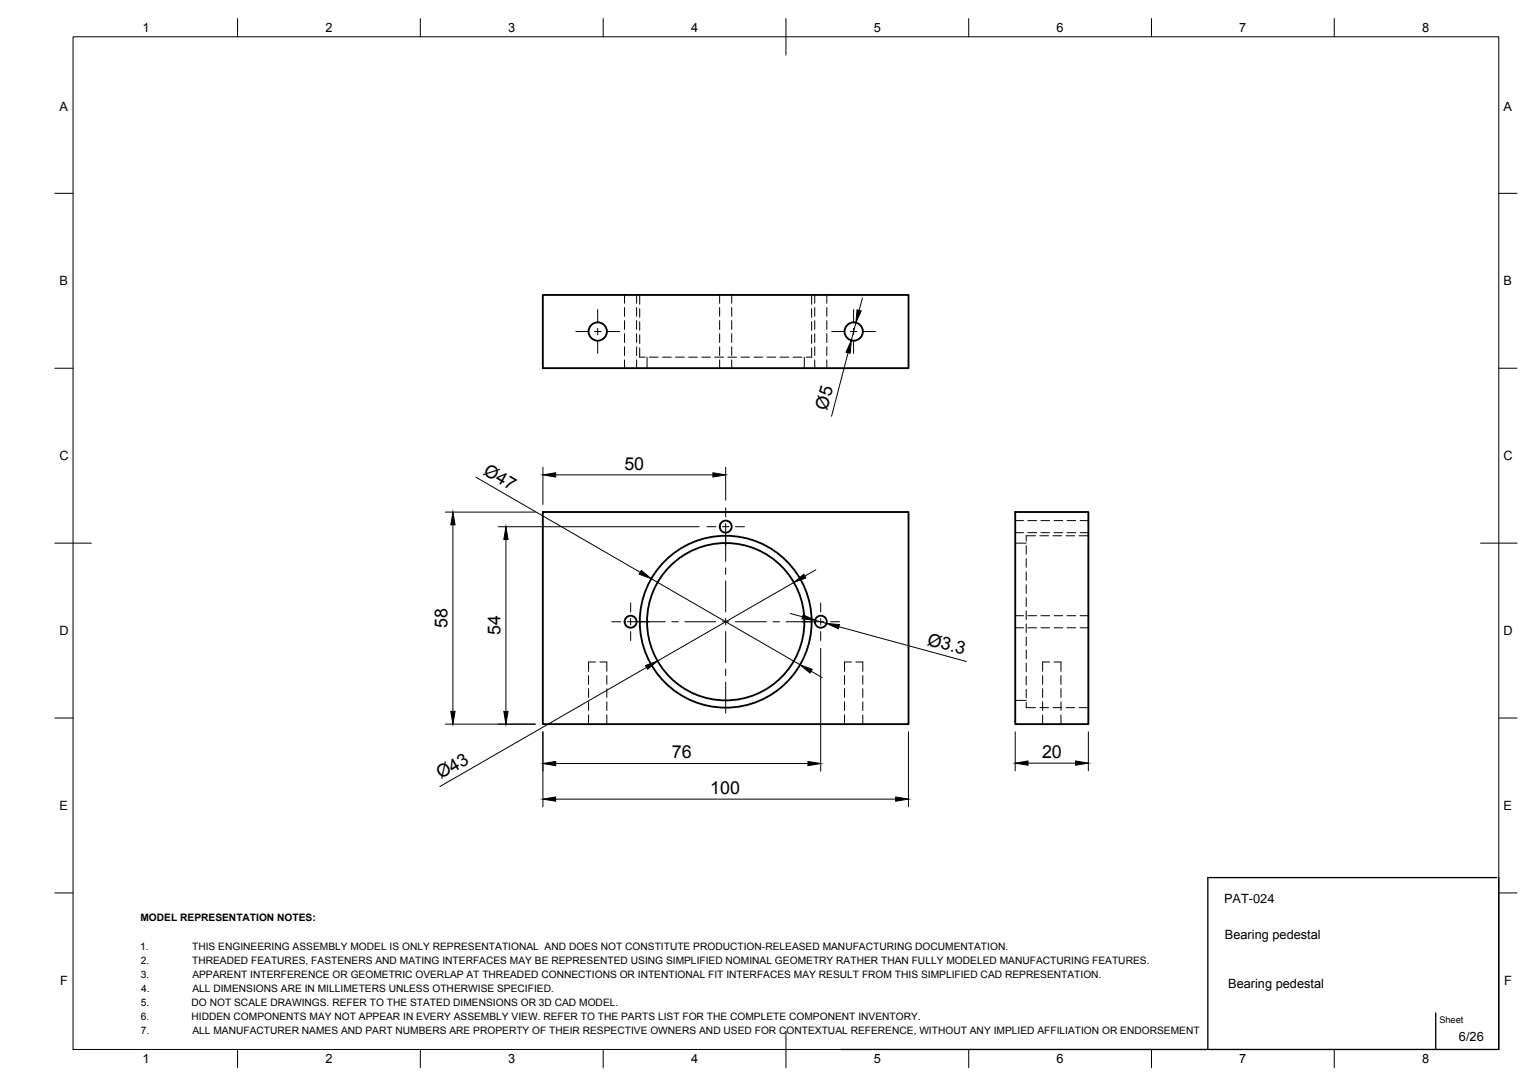
ISO-10303-21;
HEADER;
/* Generated by software containing ST-Developer
 * from STEP Tools, Inc. (www.steptools.com) 
 */

FILE_DESCRIPTION(
/* description */ ('Compact handwheel screw vise'),
/* implementation_level */ '2;1');

FILE_NAME(
/* name */ 'Bearing pedestal.step',
/* time_stamp */ '2026-10-29T16:08:22-07:00',
/* author */ (''),
/* organization */ (''),
/* preprocessor_version */ 'ST-DEVELOPER v20.2',
/* originating_system */ 'Autodesk Translation Framework v15.17.0.0',
/* authorisation */ '');

FILE_SCHEMA (('AUTOMOTIVE_DESIGN { 1 0 10303 214 3 1 1 }'));
ENDSEC;

DATA;
#10=MECHANICAL_DESIGN_GEOMETRIC_PRESENTATION_REPRESENTATION('',(#647),#25074);
#591=SHAPE_REPRESENTATION_RELATIONSHIP('SRR','None',#25199,#619);
#619=ADVANCED_BREP_SHAPE_REPRESENTATION('',(#683),#25046);
#647=STYLED_ITEM('',(#25439),#683);
#683=MANIFOLD_SOLID_BREP('Body1',#8055);
#733=FACE_BOUND('',#1547,.T.);
#734=FACE_BOUND('',#1555,.T.);
#735=FACE_BOUND('',#1556,.T.);
#736=FACE_BOUND('',#1557,.T.);
#737=FACE_BOUND('',#1558,.T.);
#738=FACE_BOUND('',#1561,.T.);
#739=FACE_BOUND('',#1562,.T.);
#740=FACE_BOUND('',#1563,.T.);
#741=FACE_BOUND('',#1564,.T.);
#742=FACE_BOUND('',#1567,.T.);
#743=FACE_BOUND('',#1568,.T.);
#847=PLANE('',#8486);
#848=PLANE('',#8493);
#849=PLANE('',#8497);
#850=PLANE('',#8498);
#851=PLANE('',#8499);
#852=PLANE('',#8500);
#853=PLANE('',#8501);
#854=PLANE('',#8502);
#855=PLANE('',#8503);
#1051=FACE_OUTER_BOUND('',#1542,.T.);
#1052=FACE_OUTER_BOUND('',#1543,.T.);
#1053=FACE_OUTER_BOUND('',#1544,.T.);
#1054=FACE_OUTER_BOUND('',#1545,.T.);
#1055=FACE_OUTER_BOUND('',#1546,.T.);
#1056=FACE_OUTER_BOUND('',#1548,.T.);
#1057=FACE_OUTER_BOUND('',#1549,.T.);
#1058=FACE_OUTER_BOUND('',#1550,.T.);
#1059=FACE_OUTER_BOUND('',#1551,.T.);
#1060=FACE_OUTER_BOUND('',#1552,.T.);
#1061=FACE_OUTER_BOUND('',#1553,.T.);
#1062=FACE_OUTER_BOUND('',#1554,.T.);
#1063=FACE_OUTER_BOUND('',#1559,.T.);
#1064=FACE_OUTER_BOUND('',#1560,.T.);
#1065=FACE_OUTER_BOUND('',#1565,.T.);
#1066=FACE_OUTER_BOUND('',#1566,.T.);
#1542=EDGE_LOOP('',(#5315,#5316,#5317,#5318));
#1543=EDGE_LOOP('',(#5319,#5320,#5321,#5322));
#1544=EDGE_LOOP('',(#5323,#5324,#5325,#5326));
#1545=EDGE_LOOP('',(#5327,#5328,#5329,#5330));
#1546=EDGE_LOOP('',(#5331));
#1547=EDGE_LOOP('',(#5332));
#1548=EDGE_LOOP('',(#5333,#5334,#5335,#5336));
#1549=EDGE_LOOP('',(#5337,#5338,#5339,#5340));
#1550=EDGE_LOOP('',(#5341));
#1551=EDGE_LOOP('',(#5342,#5343,#5344,#5345));
#1552=EDGE_LOOP('',(#5346));
#1553=EDGE_LOOP('',(#5347,#5348,#5349,#5350));
#1554=EDGE_LOOP('',(#5351,#5352,#5353,#5354));
#1555=EDGE_LOOP('',(#5355));
#1556=EDGE_LOOP('',(#5356));
#1557=EDGE_LOOP('',(#5357));
#1558=EDGE_LOOP('',(#5358));
#1559=EDGE_LOOP('',(#5359,#5360,#5361,#5362));
#1560=EDGE_LOOP('',(#5363,#5364,#5365,#5366));
#1561=EDGE_LOOP('',(#5367));
#1562=EDGE_LOOP('',(#5368));
#1563=EDGE_LOOP('',(#5369));
#1564=EDGE_LOOP('',(#5370));
#1565=EDGE_LOOP('',(#5371,#5372,#5373,#5374));
#1566=EDGE_LOOP('',(#5375,#5376,#5377,#5378));
#1567=EDGE_LOOP('',(#5379));
#1568=EDGE_LOOP('',(#5380));
#2112=LINE('',#11497,#2620);
#2113=LINE('',#11503,#2621);
#2114=LINE('',#11509,#2622);
#2115=LINE('',#11515,#2623);
#2116=LINE('',#11523,#2624);
#2117=LINE('',#11528,#2625);
#2118=LINE('',#11535,#2626);
#2119=LINE('',#11541,#2627);
#2120=LINE('',#11543,#2628);
#2121=LINE('',#11545,#2629);
#2122=LINE('',#11546,#2630);
#2123=LINE('',#11549,#2631);
#2124=LINE('',#11551,#2632);
#2125=LINE('',#11552,#2633);
#2126=LINE('',#11555,#2634);
#2127=LINE('',#11557,#2635);
#2128=LINE('',#11558,#2636);
#2129=LINE('',#11560,#2637);
#2130=LINE('',#11561,#2638);
#2620=VECTOR('',#9404,0.165);
#2621=VECTOR('',#9411,0.165);
#2622=VECTOR('',#9418,0.165);
#2623=VECTOR('',#9425,2.35);
#2624=VECTOR('',#9436,2.15);
#2625=VECTOR('',#9441,0.25);
#2626=VECTOR('',#9450,0.25);
#2627=VECTOR('',#9457,1.);
#2628=VECTOR('',#9458,1.);
#2629=VECTOR('',#9459,1.);
#2630=VECTOR('',#9460,1.);
#2631=VECTOR('',#9463,1.);
#2632=VECTOR('',#9464,1.);
#2633=VECTOR('',#9465,1.);
#2634=VECTOR('',#9468,1.);
#2635=VECTOR('',#9469,1.);
#2636=VECTOR('',#9470,1.);
#2637=VECTOR('',#9473,1.);
#2638=VECTOR('',#9474,1.);
#3106=CIRCLE('',#8475,0.165);
#3107=CIRCLE('',#8476,0.165);
#3108=CIRCLE('',#8478,0.165);
#3109=CIRCLE('',#8479,0.165);
#3110=CIRCLE('',#8481,0.165);
#3111=CIRCLE('',#8482,0.165);
#3112=CIRCLE('',#8484,2.35);
#3113=CIRCLE('',#8485,2.35);
#3114=CIRCLE('',#8487,2.15);
#3115=CIRCLE('',#8489,2.15);
#3116=CIRCLE('',#8491,0.25);
#3117=CIRCLE('',#8492,0.25);
#3118=CIRCLE('',#8495,0.25);
#3119=CIRCLE('',#8496,0.25);
#3385=VERTEX_POINT('',#11494);
#3386=VERTEX_POINT('',#11496);
#3387=VERTEX_POINT('',#11500);
#3388=VERTEX_POINT('',#11502);
#3389=VERTEX_POINT('',#11506);
#3390=VERTEX_POINT('',#11508);
#3391=VERTEX_POINT('',#11512);
#3392=VERTEX_POINT('',#11514);
#3393=VERTEX_POINT('',#11518);
#3394=VERTEX_POINT('',#11521);
#3395=VERTEX_POINT('',#11525);
#3396=VERTEX_POINT('',#11527);
#3397=VERTEX_POINT('',#11532);
#3398=VERTEX_POINT('',#11534);
#3399=VERTEX_POINT('',#11539);
#3400=VERTEX_POINT('',#11540);
#3401=VERTEX_POINT('',#11542);
#3402=VERTEX_POINT('',#11544);
#3403=VERTEX_POINT('',#11548);
#3404=VERTEX_POINT('',#11550);
#3405=VERTEX_POINT('',#11554);
#3406=VERTEX_POINT('',#11556);
#4144=EDGE_CURVE('',#3385,#3385,#3106,.T.);
#4145=EDGE_CURVE('',#3385,#3386,#2112,.T.);
#4146=EDGE_CURVE('',#3386,#3386,#3107,.T.);
#4147=EDGE_CURVE('',#3387,#3387,#3108,.T.);
#4148=EDGE_CURVE('',#3387,#3388,#2113,.T.);
#4149=EDGE_CURVE('',#3388,#3388,#3109,.T.);
#4150=EDGE_CURVE('',#3389,#3389,#3110,.T.);
#4151=EDGE_CURVE('',#3389,#3390,#2114,.T.);
#4152=EDGE_CURVE('',#3390,#3390,#3111,.T.);
#4153=EDGE_CURVE('',#3391,#3391,#3112,.T.);
#4154=EDGE_CURVE('',#3391,#3392,#2115,.T.);
#4155=EDGE_CURVE('',#3392,#3392,#3113,.T.);
#4156=EDGE_CURVE('',#3393,#3393,#3114,.T.);
#4157=EDGE_CURVE('',#3394,#3394,#3115,.T.);
#4158=EDGE_CURVE('',#3394,#3393,#2116,.T.);
#4159=EDGE_CURVE('',#3395,#3395,#3116,.T.);
#4160=EDGE_CURVE('',#3395,#3396,#2117,.T.);
#4161=EDGE_CURVE('',#3396,#3396,#3117,.T.);
#4162=EDGE_CURVE('',#3397,#3397,#3118,.T.);
#4163=EDGE_CURVE('',#3397,#3398,#2118,.T.);
#4164=EDGE_CURVE('',#3398,#3398,#3119,.T.);
#4165=EDGE_CURVE('',#3399,#3400,#2119,.T.);
#4166=EDGE_CURVE('',#3400,#3401,#2120,.T.);
#4167=EDGE_CURVE('',#3402,#3401,#2121,.T.);
#4168=EDGE_CURVE('',#3399,#3402,#2122,.T.);
#4169=EDGE_CURVE('',#3403,#3399,#2123,.T.);
#4170=EDGE_CURVE('',#3404,#3402,#2124,.T.);
#4171=EDGE_CURVE('',#3403,#3404,#2125,.T.);
#4172=EDGE_CURVE('',#3405,#3403,#2126,.T.);
#4173=EDGE_CURVE('',#3406,#3404,#2127,.T.);
#4174=EDGE_CURVE('',#3405,#3406,#2128,.T.);
#4175=EDGE_CURVE('',#3400,#3405,#2129,.T.);
#4176=EDGE_CURVE('',#3401,#3406,#2130,.T.);
#5315=ORIENTED_EDGE('',*,*,#4144,.F.);
#5316=ORIENTED_EDGE('',*,*,#4145,.T.);
#5317=ORIENTED_EDGE('',*,*,#4146,.F.);
#5318=ORIENTED_EDGE('',*,*,#4145,.F.);
#5319=ORIENTED_EDGE('',*,*,#4147,.F.);
#5320=ORIENTED_EDGE('',*,*,#4148,.T.);
#5321=ORIENTED_EDGE('',*,*,#4149,.F.);
#5322=ORIENTED_EDGE('',*,*,#4148,.F.);
#5323=ORIENTED_EDGE('',*,*,#4150,.F.);
#5324=ORIENTED_EDGE('',*,*,#4151,.T.);
#5325=ORIENTED_EDGE('',*,*,#4152,.F.);
#5326=ORIENTED_EDGE('',*,*,#4151,.F.);
#5327=ORIENTED_EDGE('',*,*,#4153,.F.);
#5328=ORIENTED_EDGE('',*,*,#4154,.T.);
#5329=ORIENTED_EDGE('',*,*,#4155,.F.);
#5330=ORIENTED_EDGE('',*,*,#4154,.F.);
#5331=ORIENTED_EDGE('',*,*,#4153,.T.);
#5332=ORIENTED_EDGE('',*,*,#4156,.F.);
#5333=ORIENTED_EDGE('',*,*,#4157,.F.);
#5334=ORIENTED_EDGE('',*,*,#4158,.T.);
#5335=ORIENTED_EDGE('',*,*,#4156,.T.);
#5336=ORIENTED_EDGE('',*,*,#4158,.F.);
#5337=ORIENTED_EDGE('',*,*,#4159,.F.);
#5338=ORIENTED_EDGE('',*,*,#4160,.T.);
#5339=ORIENTED_EDGE('',*,*,#4161,.T.);
#5340=ORIENTED_EDGE('',*,*,#4160,.F.);
#5341=ORIENTED_EDGE('',*,*,#4161,.F.);
#5342=ORIENTED_EDGE('',*,*,#4162,.F.);
#5343=ORIENTED_EDGE('',*,*,#4163,.T.);
#5344=ORIENTED_EDGE('',*,*,#4164,.T.);
#5345=ORIENTED_EDGE('',*,*,#4163,.F.);
#5346=ORIENTED_EDGE('',*,*,#4164,.F.);
#5347=ORIENTED_EDGE('',*,*,#4165,.T.);
#5348=ORIENTED_EDGE('',*,*,#4166,.T.);
#5349=ORIENTED_EDGE('',*,*,#4167,.F.);
#5350=ORIENTED_EDGE('',*,*,#4168,.F.);
#5351=ORIENTED_EDGE('',*,*,#4169,.T.);
#5352=ORIENTED_EDGE('',*,*,#4168,.T.);
#5353=ORIENTED_EDGE('',*,*,#4170,.F.);
#5354=ORIENTED_EDGE('',*,*,#4171,.F.);
#5355=ORIENTED_EDGE('',*,*,#4146,.T.);
#5356=ORIENTED_EDGE('',*,*,#4149,.T.);
#5357=ORIENTED_EDGE('',*,*,#4152,.T.);
#5358=ORIENTED_EDGE('',*,*,#4155,.T.);
#5359=ORIENTED_EDGE('',*,*,#4172,.T.);
#5360=ORIENTED_EDGE('',*,*,#4171,.T.);
#5361=ORIENTED_EDGE('',*,*,#4173,.F.);
#5362=ORIENTED_EDGE('',*,*,#4174,.F.);
#5363=ORIENTED_EDGE('',*,*,#4175,.T.);
#5364=ORIENTED_EDGE('',*,*,#4174,.T.);
#5365=ORIENTED_EDGE('',*,*,#4176,.F.);
#5366=ORIENTED_EDGE('',*,*,#4166,.F.);
#5367=ORIENTED_EDGE('',*,*,#4144,.T.);
#5368=ORIENTED_EDGE('',*,*,#4147,.T.);
#5369=ORIENTED_EDGE('',*,*,#4150,.T.);
#5370=ORIENTED_EDGE('',*,*,#4157,.T.);
#5371=ORIENTED_EDGE('',*,*,#4176,.T.);
#5372=ORIENTED_EDGE('',*,*,#4173,.T.);
#5373=ORIENTED_EDGE('',*,*,#4170,.T.);
#5374=ORIENTED_EDGE('',*,*,#4167,.T.);
#5375=ORIENTED_EDGE('',*,*,#4175,.F.);
#5376=ORIENTED_EDGE('',*,*,#4165,.F.);
#5377=ORIENTED_EDGE('',*,*,#4169,.F.);
#5378=ORIENTED_EDGE('',*,*,#4172,.F.);
#5379=ORIENTED_EDGE('',*,*,#4159,.T.);
#5380=ORIENTED_EDGE('',*,*,#4162,.T.);
#7359=CYLINDRICAL_SURFACE('',#8474,0.165);
#7360=CYLINDRICAL_SURFACE('',#8477,0.165);
#7361=CYLINDRICAL_SURFACE('',#8480,0.165);
#7362=CYLINDRICAL_SURFACE('',#8483,2.35);
#7363=CYLINDRICAL_SURFACE('',#8488,2.15);
#7364=CYLINDRICAL_SURFACE('',#8490,0.25);
#7365=CYLINDRICAL_SURFACE('',#8494,0.25);
#7621=ADVANCED_FACE('',(#1051),#7359,.F.);
#7622=ADVANCED_FACE('',(#1052),#7360,.F.);
#7623=ADVANCED_FACE('',(#1053),#7361,.F.);
#7624=ADVANCED_FACE('',(#1054),#7362,.F.);
#7625=ADVANCED_FACE('',(#1055,#733),#847,.T.);
#7626=ADVANCED_FACE('',(#1056),#7363,.F.);
#7627=ADVANCED_FACE('',(#1057),#7364,.F.);
#7628=ADVANCED_FACE('',(#1058),#848,.F.);
#7629=ADVANCED_FACE('',(#1059),#7365,.F.);
#7630=ADVANCED_FACE('',(#1060),#849,.F.);
#7631=ADVANCED_FACE('',(#1061),#850,.T.);
#7632=ADVANCED_FACE('',(#1062,#734,#735,#736,#737),#851,.T.);
#7633=ADVANCED_FACE('',(#1063),#852,.T.);
#7634=ADVANCED_FACE('',(#1064,#738,#739,#740,#741),#853,.T.);
#7635=ADVANCED_FACE('',(#1065),#854,.T.);
#7636=ADVANCED_FACE('',(#1066,#742,#743),#855,.F.);
#8055=CLOSED_SHELL('',(#7621,#7622,#7623,#7624,#7625,#7626,#7627,#7628,
#7629,#7630,#7631,#7632,#7633,#7634,#7635,#7636));
#8473=AXIS2_PLACEMENT_3D('',#11492,#9398,#9399);
#8474=AXIS2_PLACEMENT_3D('',#11493,#9400,#9401);
#8475=AXIS2_PLACEMENT_3D('',#11495,#9402,#9403);
#8476=AXIS2_PLACEMENT_3D('',#11498,#9405,#9406);
#8477=AXIS2_PLACEMENT_3D('',#11499,#9407,#9408);
#8478=AXIS2_PLACEMENT_3D('',#11501,#9409,#9410);
#8479=AXIS2_PLACEMENT_3D('',#11504,#9412,#9413);
#8480=AXIS2_PLACEMENT_3D('',#11505,#9414,#9415);
#8481=AXIS2_PLACEMENT_3D('',#11507,#9416,#9417);
#8482=AXIS2_PLACEMENT_3D('',#11510,#9419,#9420);
#8483=AXIS2_PLACEMENT_3D('',#11511,#9421,#9422);
#8484=AXIS2_PLACEMENT_3D('',#11513,#9423,#9424);
#8485=AXIS2_PLACEMENT_3D('',#11516,#9426,#9427);
#8486=AXIS2_PLACEMENT_3D('',#11517,#9428,#9429);
#8487=AXIS2_PLACEMENT_3D('',#11519,#9430,#9431);
#8488=AXIS2_PLACEMENT_3D('',#11520,#9432,#9433);
#8489=AXIS2_PLACEMENT_3D('',#11522,#9434,#9435);
#8490=AXIS2_PLACEMENT_3D('',#11524,#9437,#9438);
#8491=AXIS2_PLACEMENT_3D('',#11526,#9439,#9440);
#8492=AXIS2_PLACEMENT_3D('',#11529,#9442,#9443);
#8493=AXIS2_PLACEMENT_3D('',#11530,#9444,#9445);
#8494=AXIS2_PLACEMENT_3D('',#11531,#9446,#9447);
#8495=AXIS2_PLACEMENT_3D('',#11533,#9448,#9449);
#8496=AXIS2_PLACEMENT_3D('',#11536,#9451,#9452);
#8497=AXIS2_PLACEMENT_3D('',#11537,#9453,#9454);
#8498=AXIS2_PLACEMENT_3D('',#11538,#9455,#9456);
#8499=AXIS2_PLACEMENT_3D('',#11547,#9461,#9462);
#8500=AXIS2_PLACEMENT_3D('',#11553,#9466,#9467);
#8501=AXIS2_PLACEMENT_3D('',#11559,#9471,#9472);
#8502=AXIS2_PLACEMENT_3D('',#11562,#9475,#9476);
#8503=AXIS2_PLACEMENT_3D('',#11563,#9477,#9478);
#9398=DIRECTION('axis',(0.,0.,1.));
#9399=DIRECTION('refdir',(1.,0.,0.));
#9400=DIRECTION('center_axis',(1.,0.,0.));
#9401=DIRECTION('ref_axis',(0.,0.,-1.));
#9402=DIRECTION('center_axis',(1.,0.,0.));
#9403=DIRECTION('ref_axis',(0.,0.,-1.));
#9404=DIRECTION('',(1.,0.,0.));
#9405=DIRECTION('center_axis',(-1.,0.,0.));
#9406=DIRECTION('ref_axis',(0.,0.,-1.));
#9407=DIRECTION('center_axis',(1.,0.,0.));
#9408=DIRECTION('ref_axis',(0.,0.,-1.));
#9409=DIRECTION('center_axis',(1.,0.,0.));
#9410=DIRECTION('ref_axis',(0.,0.,-1.));
#9411=DIRECTION('',(1.,0.,0.));
#9412=DIRECTION('center_axis',(-1.,0.,0.));
#9413=DIRECTION('ref_axis',(0.,0.,-1.));
#9414=DIRECTION('center_axis',(1.,0.,0.));
#9415=DIRECTION('ref_axis',(0.,0.,-1.));
#9416=DIRECTION('center_axis',(1.,0.,0.));
#9417=DIRECTION('ref_axis',(0.,0.,-1.));
#9418=DIRECTION('',(1.,0.,0.));
#9419=DIRECTION('center_axis',(-1.,0.,0.));
#9420=DIRECTION('ref_axis',(0.,0.,-1.));
#9421=DIRECTION('center_axis',(1.,0.,0.));
#9422=DIRECTION('ref_axis',(0.,0.,-1.));
#9423=DIRECTION('center_axis',(1.,0.,0.));
#9424=DIRECTION('ref_axis',(0.,0.,-1.));
#9425=DIRECTION('',(1.,0.,0.));
#9426=DIRECTION('center_axis',(-1.,0.,0.));
#9427=DIRECTION('ref_axis',(0.,0.,-1.));
#9428=DIRECTION('center_axis',(1.,0.,0.));
#9429=DIRECTION('ref_axis',(0.,0.,-1.));
#9430=DIRECTION('center_axis',(1.,0.,0.));
#9431=DIRECTION('ref_axis',(0.,0.,-1.));
#9432=DIRECTION('center_axis',(1.,0.,0.));
#9433=DIRECTION('ref_axis',(0.,0.,-1.));
#9434=DIRECTION('center_axis',(1.,0.,0.));
#9435=DIRECTION('ref_axis',(0.,0.,-1.));
#9436=DIRECTION('',(1.,0.,0.));
#9437=DIRECTION('center_axis',(0.,0.,1.));
#9438=DIRECTION('ref_axis',(1.,0.,0.));
#9439=DIRECTION('center_axis',(0.,0.,1.));
#9440=DIRECTION('ref_axis',(1.,0.,0.));
#9441=DIRECTION('',(0.,0.,1.));
#9442=DIRECTION('center_axis',(0.,0.,1.));
#9443=DIRECTION('ref_axis',(1.,0.,0.));
#9444=DIRECTION('center_axis',(0.,0.,1.));
#9445=DIRECTION('ref_axis',(1.,0.,0.));
#9446=DIRECTION('center_axis',(0.,0.,1.));
#9447=DIRECTION('ref_axis',(1.,0.,0.));
#9448=DIRECTION('center_axis',(0.,0.,1.));
#9449=DIRECTION('ref_axis',(1.,0.,0.));
#9450=DIRECTION('',(0.,0.,1.));
#9451=DIRECTION('center_axis',(0.,0.,1.));
#9452=DIRECTION('ref_axis',(1.,0.,0.));
#9453=DIRECTION('center_axis',(0.,0.,1.));
#9454=DIRECTION('ref_axis',(1.,0.,0.));
#9455=DIRECTION('center_axis',(0.,1.,0.));
#9456=DIRECTION('ref_axis',(-1.,0.,0.));
#9457=DIRECTION('',(-1.,0.,0.));
#9458=DIRECTION('',(0.,0.,1.));
#9459=DIRECTION('',(-1.,0.,0.));
#9460=DIRECTION('',(0.,0.,1.));
#9461=DIRECTION('center_axis',(1.,0.,0.));
#9462=DIRECTION('ref_axis',(0.,1.,0.));
#9463=DIRECTION('',(0.,1.,0.));
#9464=DIRECTION('',(0.,1.,0.));
#9465=DIRECTION('',(0.,0.,1.));
#9466=DIRECTION('center_axis',(0.,-1.,0.));
#9467=DIRECTION('ref_axis',(1.,0.,0.));
#9468=DIRECTION('',(1.,0.,0.));
#9469=DIRECTION('',(1.,0.,0.));
#9470=DIRECTION('',(0.,0.,1.));
#9471=DIRECTION('center_axis',(-1.,0.,0.));
#9472=DIRECTION('ref_axis',(0.,-1.,0.));
#9473=DIRECTION('',(0.,-1.,0.));
#9474=DIRECTION('',(0.,-1.,0.));
#9475=DIRECTION('center_axis',(0.,0.,1.));
#9476=DIRECTION('ref_axis',(1.,0.,0.));
#9477=DIRECTION('center_axis',(0.,0.,1.));
#9478=DIRECTION('ref_axis',(1.,0.,0.));
#11492=CARTESIAN_POINT('',(0.,0.,0.));
#11493=CARTESIAN_POINT('Origin',(22.9,2.6,4.));
#11494=CARTESIAN_POINT('',(23.,2.6,4.165));
#11495=CARTESIAN_POINT('Origin',(23.,2.6,4.));
#11496=CARTESIAN_POINT('',(25.,2.6,4.165));
#11497=CARTESIAN_POINT('',(22.9,2.6,4.165));
#11498=CARTESIAN_POINT('Origin',(25.,2.6,4.));
#11499=CARTESIAN_POINT('Origin',(22.9,1.59204083889156E-16,6.6));
#11500=CARTESIAN_POINT('',(23.,1.38997411703225E-16,6.765));
#11501=CARTESIAN_POINT('Origin',(23.,1.59204083889156E-16,6.6));
#11502=CARTESIAN_POINT('',(25.,1.79410756075087E-16,6.765));
#11503=CARTESIAN_POINT('',(22.9,1.38997411703225E-16,6.765));
#11504=CARTESIAN_POINT('Origin',(25.,1.59204083889156E-16,6.6));
#11505=CARTESIAN_POINT('Origin',(22.9,-2.6,4.));
#11506=CARTESIAN_POINT('',(23.,-2.6,4.165));
#11507=CARTESIAN_POINT('Origin',(23.,-2.6,4.));
#11508=CARTESIAN_POINT('',(25.,-2.6,4.165));
#11509=CARTESIAN_POINT('',(22.9,-2.6,4.165));
#11510=CARTESIAN_POINT('Origin',(25.,-2.6,4.));
#11511=CARTESIAN_POINT('Origin',(23.3,0.,4.));
#11512=CARTESIAN_POINT('',(23.3,-2.87791997799628E-16,6.35));
#11513=CARTESIAN_POINT('Origin',(23.3,0.,4.));
#11514=CARTESIAN_POINT('',(25.,2.87791997799628E-16,6.35));
#11515=CARTESIAN_POINT('',(23.3,-2.87791997799628E-16,6.35));
#11516=CARTESIAN_POINT('Origin',(25.,0.,4.));
#11517=CARTESIAN_POINT('Origin',(23.3,0.,4.));
#11518=CARTESIAN_POINT('',(23.3,-2.63299061816681E-16,6.15));
#11519=CARTESIAN_POINT('Origin',(23.3,0.,4.));
#11520=CARTESIAN_POINT('Origin',(22.9,0.,4.));
#11521=CARTESIAN_POINT('',(23.,-2.63299061816681E-16,6.15));
#11522=CARTESIAN_POINT('Origin',(23.,0.,4.));
#11523=CARTESIAN_POINT('',(22.9,-2.63299061816681E-16,6.15));
#11524=CARTESIAN_POINT('Origin',(24.,-3.5,1.1));
#11525=CARTESIAN_POINT('',(23.75,-3.5,1.2));
#11526=CARTESIAN_POINT('Origin',(24.,-3.5,1.2));
#11527=CARTESIAN_POINT('',(23.75,-3.5,2.9));
#11528=CARTESIAN_POINT('',(23.75,-3.5,1.1));
#11529=CARTESIAN_POINT('Origin',(24.,-3.5,2.9));
#11530=CARTESIAN_POINT('Origin',(24.,-3.5,2.9));
#11531=CARTESIAN_POINT('Origin',(24.,3.5,1.1));
#11532=CARTESIAN_POINT('',(23.75,3.5,1.2));
#11533=CARTESIAN_POINT('Origin',(24.,3.5,1.2));
#11534=CARTESIAN_POINT('',(23.75,3.5,2.9));
#11535=CARTESIAN_POINT('',(23.75,3.5,1.1));
#11536=CARTESIAN_POINT('Origin',(24.,3.5,2.9));
#11537=CARTESIAN_POINT('Origin',(24.,3.5,2.9));
#11538=CARTESIAN_POINT('Origin',(25.,5.,1.2));
#11539=CARTESIAN_POINT('',(25.,5.,1.2));
#11540=CARTESIAN_POINT('',(23.,5.,1.2));
#11541=CARTESIAN_POINT('',(25.,5.,1.2));
#11542=CARTESIAN_POINT('',(23.,5.,7.));
#11543=CARTESIAN_POINT('',(23.,5.,1.2));
#11544=CARTESIAN_POINT('',(25.,5.,7.));
#11545=CARTESIAN_POINT('',(25.,5.,7.));
#11546=CARTESIAN_POINT('',(25.,5.,1.2));
#11547=CARTESIAN_POINT('Origin',(25.,-5.,1.2));
#11548=CARTESIAN_POINT('',(25.,-5.,1.2));
#11549=CARTESIAN_POINT('',(25.,-5.,1.2));
#11550=CARTESIAN_POINT('',(25.,-5.,7.));
#11551=CARTESIAN_POINT('',(25.,-5.,7.));
#11552=CARTESIAN_POINT('',(25.,-5.,1.2));
#11553=CARTESIAN_POINT('Origin',(23.,-5.,1.2));
#11554=CARTESIAN_POINT('',(23.,-5.,1.2));
#11555=CARTESIAN_POINT('',(23.,-5.,1.2));
#11556=CARTESIAN_POINT('',(23.,-5.,7.));
#11557=CARTESIAN_POINT('',(23.,-5.,7.));
#11558=CARTESIAN_POINT('',(23.,-5.,1.2));
#11559=CARTESIAN_POINT('Origin',(23.,5.,1.2));
#11560=CARTESIAN_POINT('',(23.,5.,1.2));
#11561=CARTESIAN_POINT('',(23.,5.,7.));
#11562=CARTESIAN_POINT('Origin',(24.,0.,7.));
#11563=CARTESIAN_POINT('Origin',(24.,0.,1.2));
#25012=UNCERTAINTY_MEASURE_WITH_UNIT(LENGTH_MEASURE(0.001),#25075,
'DISTANCE_ACCURACY_VALUE',
'Maximum model space distance between geometric entities at asserted c
onnectivities');
#25040=UNCERTAINTY_MEASURE_WITH_UNIT(LENGTH_MEASURE(0.001),#25075,
'DISTANCE_ACCURACY_VALUE',
'Maximum model space distance between geometric entities at asserted c
onnectivities');
#25046=(
GEOMETRIC_REPRESENTATION_CONTEXT(3)
GLOBAL_UNCERTAINTY_ASSIGNED_CONTEXT((#25012))
GLOBAL_UNIT_ASSIGNED_CONTEXT((#25075,#25077,#25078))
REPRESENTATION_CONTEXT('','3D')
);
#25074=(
GEOMETRIC_REPRESENTATION_CONTEXT(3)
GLOBAL_UNCERTAINTY_ASSIGNED_CONTEXT((#25040))
GLOBAL_UNIT_ASSIGNED_CONTEXT((#25075,#25077,#25078))
REPRESENTATION_CONTEXT('','3D')
);
#25075=(
LENGTH_UNIT()
NAMED_UNIT(*)
SI_UNIT(.CENTI.,.METRE.)
);
#25077=(
NAMED_UNIT(*)
PLANE_ANGLE_UNIT()
SI_UNIT($,.RADIAN.)
);
#25078=(
NAMED_UNIT(*)
SI_UNIT($,.STERADIAN.)
SOLID_ANGLE_UNIT()
);
#25084=SHAPE_DEFINITION_REPRESENTATION(#25117,#25199);
#25117=PRODUCT_DEFINITION_SHAPE('',$,#25233);
#25199=SHAPE_REPRESENTATION('',(#8473),#25046);
#25227=PRODUCT_DEFINITION_CONTEXT('part definition',#25328,'design');
#25233=PRODUCT_DEFINITION('Bearing pedestal','Bearing pedestal',#25266,
#25227);
#25266=PRODUCT_DEFINITION_FORMATION('',$,#25335);
#25328=APPLICATION_CONTEXT(
'Core Data for Automotive Mechanical Design Process');
#25329=PRODUCT_CONTEXT('part definition',#25328,'mechanical');
#25335=PRODUCT('Bearing pedestal','Bearing pedestal','Bearing pedestal',
(#25329));
#25433=COLOUR_RGB('Grey',0.48,0.52,0.57);
#25434=FILL_AREA_STYLE_COLOUR('',#25433);
#25435=FILL_AREA_STYLE('',(#25434));
#25436=SURFACE_STYLE_FILL_AREA(#25435);
#25437=SURFACE_SIDE_STYLE('',(#25436));
#25438=SURFACE_STYLE_USAGE(.BOTH.,#25437);
#25439=PRESENTATION_STYLE_ASSIGNMENT((#25438));
ENDSEC;
END-ISO-10303-21;
